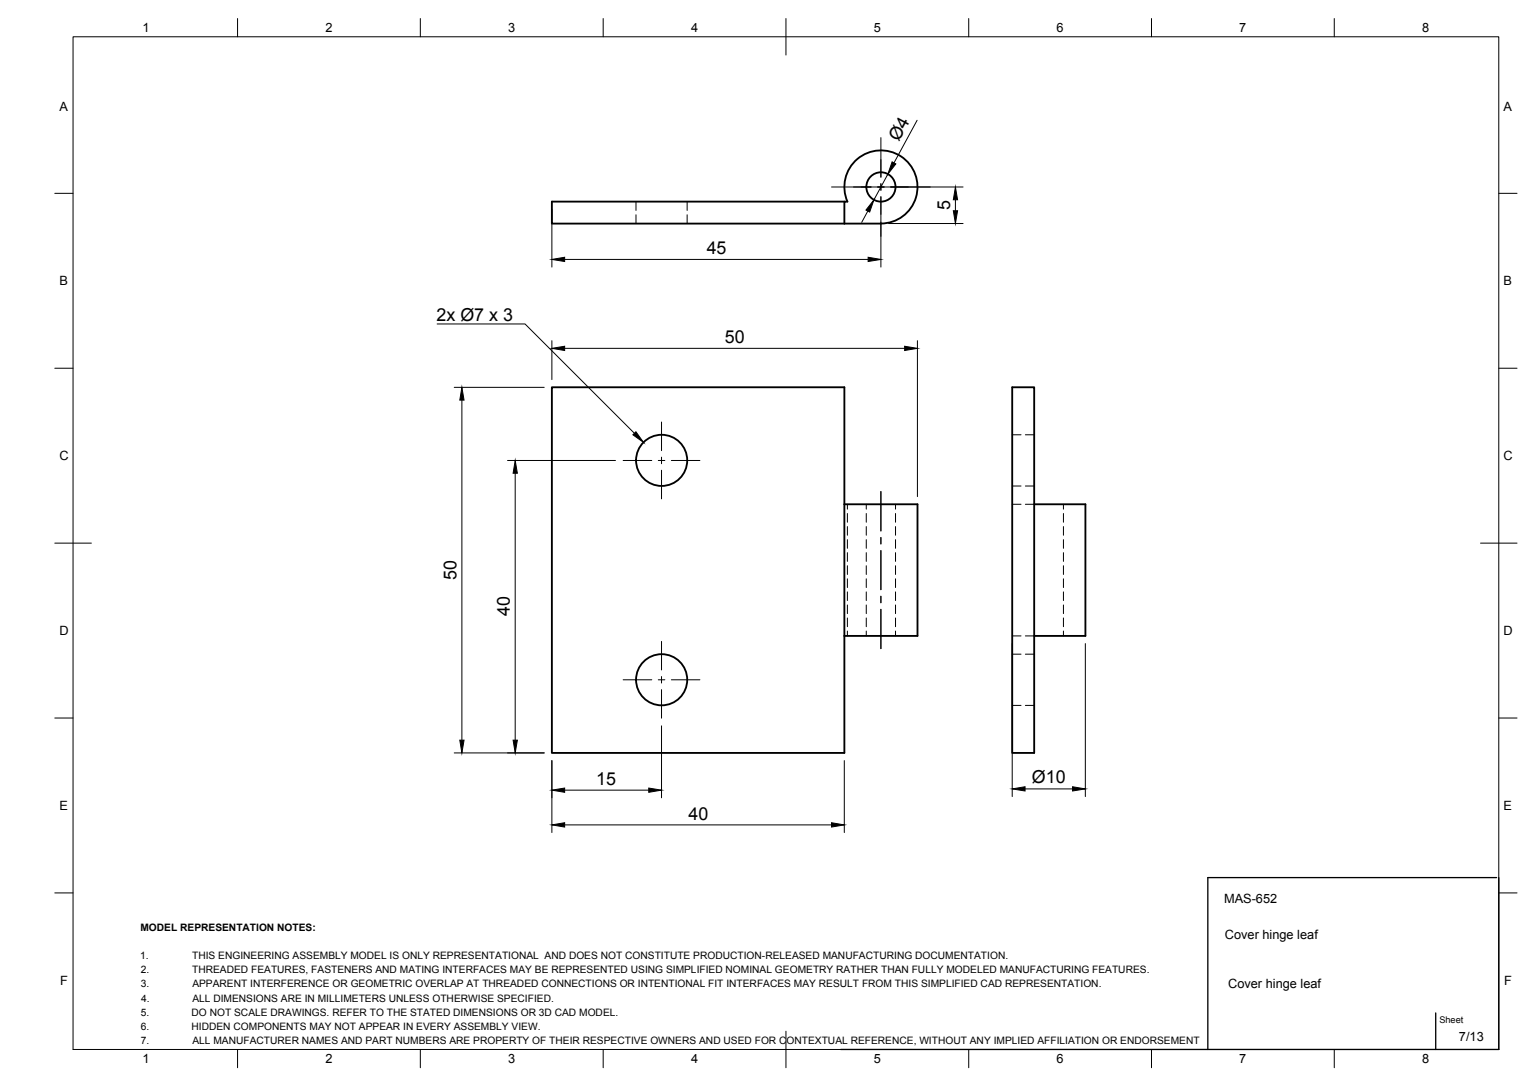
ISO-10303-21;
HEADER;
/* Generated by software containing ST-Developer
 * from STEP Tools, Inc. (www.steptools.com) 
 */

FILE_DESCRIPTION(
/* description */ ('Independent hinged machine back cover with retained hinge pins, perim
eter gasket and quarter-turn cam latch. Nominal cover 360 x 260 x 3 mm
, frame 430 x 300 x 20 mm. No guarding, structural or ingress rating a
ssigned.'),
/* implementation_level */ '2;1');

FILE_NAME(
/* name */ 'Cover hinge leaf.step',
/* time_stamp */ '2026-11-09T19:36:59-08:00',
/* author */ (''),
/* organization */ (''),
/* preprocessor_version */ 'ST-DEVELOPER v20.2',
/* originating_system */ 'Autodesk Translation Framework v15.17.0.0',
/* authorisation */ '');

FILE_SCHEMA (('AUTOMOTIVE_DESIGN { 1 0 10303 214 3 1 1 }'));
ENDSEC;

DATA;
#10=MECHANICAL_DESIGN_GEOMETRIC_PRESENTATION_REPRESENTATION('',(#210),#32627);
#174=SHAPE_REPRESENTATION_RELATIONSHIP('SRR','None',#32720,#192);
#192=ADVANCED_BREP_SHAPE_REPRESENTATION('',(#228),#32621);
#210=STYLED_ITEM('',(#32811),#228);
#228=MANIFOLD_SOLID_BREP('Body1',#8687);
#277=FACE_BOUND('',#1313,.T.);
#278=FACE_BOUND('',#1314,.T.);
#279=FACE_BOUND('',#1319,.T.);
#280=FACE_BOUND('',#1323,.T.);
#281=FACE_BOUND('',#1327,.T.);
#282=FACE_BOUND('',#1328,.T.);
#411=PLANE('',#9324);
#412=PLANE('',#9325);
#413=PLANE('',#9326);
#414=PLANE('',#9329);
#415=PLANE('',#9334);
#416=PLANE('',#9341);
#417=PLANE('',#9342);
#418=PLANE('',#9343);
#419=PLANE('',#9344);
#792=FACE_OUTER_BOUND('',#1310,.T.);
#793=FACE_OUTER_BOUND('',#1311,.T.);
#794=FACE_OUTER_BOUND('',#1312,.T.);
#795=FACE_OUTER_BOUND('',#1315,.T.);
#796=FACE_OUTER_BOUND('',#1316,.T.);
#797=FACE_OUTER_BOUND('',#1317,.T.);
#798=FACE_OUTER_BOUND('',#1318,.T.);
#799=FACE_OUTER_BOUND('',#1320,.T.);
#800=FACE_OUTER_BOUND('',#1321,.T.);
#801=FACE_OUTER_BOUND('',#1322,.T.);
#802=FACE_OUTER_BOUND('',#1324,.T.);
#803=FACE_OUTER_BOUND('',#1325,.T.);
#804=FACE_OUTER_BOUND('',#1326,.T.);
#1310=EDGE_LOOP('',(#7173,#7174,#7175,#7176));
#1311=EDGE_LOOP('',(#7177,#7178,#7179,#7180));
#1312=EDGE_LOOP('',(#7181,#7182,#7183,#7184,#7185,#7186,#7187,#7188));
#1313=EDGE_LOOP('',(#7189));
#1314=EDGE_LOOP('',(#7190));
#1315=EDGE_LOOP('',(#7191,#7192,#7193,#7194));
#1316=EDGE_LOOP('',(#7195,#7196,#7197,#7198));
#1317=EDGE_LOOP('',(#7199,#7200,#7201,#7202));
#1318=EDGE_LOOP('',(#7203,#7204,#7205,#7206));
#1319=EDGE_LOOP('',(#7207));
#1320=EDGE_LOOP('',(#7208,#7209,#7210,#7211));
#1321=EDGE_LOOP('',(#7212,#7213,#7214,#7215));
#1322=EDGE_LOOP('',(#7216,#7217,#7218,#7219));
#1323=EDGE_LOOP('',(#7220));
#1324=EDGE_LOOP('',(#7221,#7222,#7223,#7224));
#1325=EDGE_LOOP('',(#7225,#7226,#7227,#7228));
#1326=EDGE_LOOP('',(#7229,#7230,#7231,#7232,#7233,#7234,#7235,#7236));
#1327=EDGE_LOOP('',(#7237));
#1328=EDGE_LOOP('',(#7238));
#1551=CIRCLE('',#9327,3.5);
#1552=CIRCLE('',#9328,3.5);
#1553=CIRCLE('',#9331,3.5);
#1554=CIRCLE('',#9333,3.5);
#1555=CIRCLE('',#9335,5.);
#1556=CIRCLE('',#9336,2.);
#1557=CIRCLE('',#9338,2.);
#1558=CIRCLE('',#9340,5.);
#2564=LINE('',#26316,#3110);
#2565=LINE('',#26318,#3111);
#2566=LINE('',#26320,#3112);
#2567=LINE('',#26321,#3113);
#2568=LINE('',#26325,#3114);
#2569=LINE('',#26327,#3115);
#2570=LINE('',#26329,#3116);
#2571=LINE('',#26330,#3117);
#2572=LINE('',#26333,#3118);
#2573=LINE('',#26335,#3119);
#2574=LINE('',#26336,#3120);
#2575=LINE('',#26338,#3121);
#2576=LINE('',#26340,#3122);
#2577=LINE('',#26341,#3123);
#2578=LINE('',#26348,#3124);
#2579=LINE('',#26349,#3125);
#2580=LINE('',#26353,#3126);
#2581=LINE('',#26357,#3127);
#2582=LINE('',#26361,#3128);
#2583=LINE('',#26366,#3129);
#2584=LINE('',#26370,#3130);
#2585=LINE('',#26373,#3131);
#2586=LINE('',#26376,#3132);
#2587=LINE('',#26377,#3133);
#2588=LINE('',#26379,#3134);
#3110=VECTOR('',#10784,10.);
#3111=VECTOR('',#10785,10.);
#3112=VECTOR('',#10786,10.);
#3113=VECTOR('',#10787,10.);
#3114=VECTOR('',#10790,10.);
#3115=VECTOR('',#10791,10.);
#3116=VECTOR('',#10792,10.);
#3117=VECTOR('',#10793,10.);
#3118=VECTOR('',#10796,10.);
#3119=VECTOR('',#10797,10.);
#3120=VECTOR('',#10798,10.);
#3121=VECTOR('',#10799,10.);
#3122=VECTOR('',#10800,10.);
#3123=VECTOR('',#10801,10.);
#3124=VECTOR('',#10808,10.);
#3125=VECTOR('',#10809,10.);
#3126=VECTOR('',#10814,3.5);
#3127=VECTOR('',#10819,3.5);
#3128=VECTOR('',#10824,10.);
#3129=VECTOR('',#10829,2.);
#3130=VECTOR('',#10834,10.);
#3131=VECTOR('',#10839,10.);
#3132=VECTOR('',#10842,10.);
#3133=VECTOR('',#10843,10.);
#3134=VECTOR('',#10846,10.);
#3869=VERTEX_POINT('',#26314);
#3870=VERTEX_POINT('',#26315);
#3871=VERTEX_POINT('',#26317);
#3872=VERTEX_POINT('',#26319);
#3873=VERTEX_POINT('',#26323);
#3874=VERTEX_POINT('',#26324);
#3875=VERTEX_POINT('',#26326);
#3876=VERTEX_POINT('',#26328);
#3877=VERTEX_POINT('',#26332);
#3878=VERTEX_POINT('',#26334);
#3879=VERTEX_POINT('',#26337);
#3880=VERTEX_POINT('',#26339);
#3881=VERTEX_POINT('',#26342);
#3882=VERTEX_POINT('',#26344);
#3883=VERTEX_POINT('',#26347);
#3884=VERTEX_POINT('',#26351);
#3885=VERTEX_POINT('',#26355);
#3886=VERTEX_POINT('',#26359);
#3887=VERTEX_POINT('',#26362);
#3888=VERTEX_POINT('',#26365);
#3889=VERTEX_POINT('',#26369);
#3890=VERTEX_POINT('',#26375);
#5010=EDGE_CURVE('',#3869,#3870,#2564,.T.);
#5011=EDGE_CURVE('',#3869,#3871,#2565,.T.);
#5012=EDGE_CURVE('',#3872,#3871,#2566,.T.);
#5013=EDGE_CURVE('',#3870,#3872,#2567,.T.);
#5014=EDGE_CURVE('',#3873,#3874,#2568,.T.);
#5015=EDGE_CURVE('',#3875,#3873,#2569,.T.);
#5016=EDGE_CURVE('',#3876,#3875,#2570,.T.);
#5017=EDGE_CURVE('',#3874,#3876,#2571,.T.);
#5018=EDGE_CURVE('',#3871,#3877,#2572,.T.);
#5019=EDGE_CURVE('',#3877,#3878,#2573,.T.);
#5020=EDGE_CURVE('',#3878,#3876,#2574,.T.);
#5021=EDGE_CURVE('',#3879,#3875,#2575,.T.);
#5022=EDGE_CURVE('',#3880,#3879,#2576,.T.);
#5023=EDGE_CURVE('',#3872,#3880,#2577,.T.);
#5024=EDGE_CURVE('',#3881,#3881,#1551,.T.);
#5025=EDGE_CURVE('',#3882,#3882,#1552,.T.);
#5026=EDGE_CURVE('',#3883,#3873,#2578,.T.);
#5027=EDGE_CURVE('',#3879,#3883,#2579,.T.);
#5028=EDGE_CURVE('',#3884,#3884,#1553,.T.);
#5029=EDGE_CURVE('',#3884,#3882,#2580,.T.);
#5030=EDGE_CURVE('',#3885,#3885,#1554,.T.);
#5031=EDGE_CURVE('',#3885,#3881,#2581,.T.);
#5032=EDGE_CURVE('',#3878,#3886,#1555,.T.);
#5033=EDGE_CURVE('',#3874,#3886,#2582,.T.);
#5034=EDGE_CURVE('',#3887,#3887,#1556,.T.);
#5035=EDGE_CURVE('',#3887,#3888,#2583,.T.);
#5036=EDGE_CURVE('',#3888,#3888,#1557,.T.);
#5037=EDGE_CURVE('',#3886,#3889,#2584,.T.);
#5038=EDGE_CURVE('',#3877,#3889,#1558,.T.);
#5039=EDGE_CURVE('',#3889,#3869,#2585,.T.);
#5040=EDGE_CURVE('',#3890,#3883,#2586,.T.);
#5041=EDGE_CURVE('',#3880,#3890,#2587,.T.);
#5042=EDGE_CURVE('',#3870,#3890,#2588,.T.);
#7173=ORIENTED_EDGE('',*,*,#5010,.F.);
#7174=ORIENTED_EDGE('',*,*,#5011,.T.);
#7175=ORIENTED_EDGE('',*,*,#5012,.F.);
#7176=ORIENTED_EDGE('',*,*,#5013,.F.);
#7177=ORIENTED_EDGE('',*,*,#5014,.F.);
#7178=ORIENTED_EDGE('',*,*,#5015,.F.);
#7179=ORIENTED_EDGE('',*,*,#5016,.F.);
#7180=ORIENTED_EDGE('',*,*,#5017,.F.);
#7181=ORIENTED_EDGE('',*,*,#5012,.T.);
#7182=ORIENTED_EDGE('',*,*,#5018,.T.);
#7183=ORIENTED_EDGE('',*,*,#5019,.T.);
#7184=ORIENTED_EDGE('',*,*,#5020,.T.);
#7185=ORIENTED_EDGE('',*,*,#5016,.T.);
#7186=ORIENTED_EDGE('',*,*,#5021,.F.);
#7187=ORIENTED_EDGE('',*,*,#5022,.F.);
#7188=ORIENTED_EDGE('',*,*,#5023,.F.);
#7189=ORIENTED_EDGE('',*,*,#5024,.T.);
#7190=ORIENTED_EDGE('',*,*,#5025,.T.);
#7191=ORIENTED_EDGE('',*,*,#5015,.T.);
#7192=ORIENTED_EDGE('',*,*,#5026,.F.);
#7193=ORIENTED_EDGE('',*,*,#5027,.F.);
#7194=ORIENTED_EDGE('',*,*,#5021,.T.);
#7195=ORIENTED_EDGE('',*,*,#5028,.F.);
#7196=ORIENTED_EDGE('',*,*,#5029,.T.);
#7197=ORIENTED_EDGE('',*,*,#5025,.F.);
#7198=ORIENTED_EDGE('',*,*,#5029,.F.);
#7199=ORIENTED_EDGE('',*,*,#5030,.F.);
#7200=ORIENTED_EDGE('',*,*,#5031,.T.);
#7201=ORIENTED_EDGE('',*,*,#5024,.F.);
#7202=ORIENTED_EDGE('',*,*,#5031,.F.);
#7203=ORIENTED_EDGE('',*,*,#5032,.T.);
#7204=ORIENTED_EDGE('',*,*,#5033,.F.);
#7205=ORIENTED_EDGE('',*,*,#5017,.T.);
#7206=ORIENTED_EDGE('',*,*,#5020,.F.);
#7207=ORIENTED_EDGE('',*,*,#5034,.T.);
#7208=ORIENTED_EDGE('',*,*,#5034,.F.);
#7209=ORIENTED_EDGE('',*,*,#5035,.T.);
#7210=ORIENTED_EDGE('',*,*,#5036,.T.);
#7211=ORIENTED_EDGE('',*,*,#5035,.F.);
#7212=ORIENTED_EDGE('',*,*,#5037,.F.);
#7213=ORIENTED_EDGE('',*,*,#5032,.F.);
#7214=ORIENTED_EDGE('',*,*,#5019,.F.);
#7215=ORIENTED_EDGE('',*,*,#5038,.T.);
#7216=ORIENTED_EDGE('',*,*,#5018,.F.);
#7217=ORIENTED_EDGE('',*,*,#5011,.F.);
#7218=ORIENTED_EDGE('',*,*,#5039,.F.);
#7219=ORIENTED_EDGE('',*,*,#5038,.F.);
#7220=ORIENTED_EDGE('',*,*,#5036,.F.);
#7221=ORIENTED_EDGE('',*,*,#5022,.T.);
#7222=ORIENTED_EDGE('',*,*,#5027,.T.);
#7223=ORIENTED_EDGE('',*,*,#5040,.F.);
#7224=ORIENTED_EDGE('',*,*,#5041,.F.);
#7225=ORIENTED_EDGE('',*,*,#5013,.T.);
#7226=ORIENTED_EDGE('',*,*,#5023,.T.);
#7227=ORIENTED_EDGE('',*,*,#5041,.T.);
#7228=ORIENTED_EDGE('',*,*,#5042,.F.);
#7229=ORIENTED_EDGE('',*,*,#5010,.T.);
#7230=ORIENTED_EDGE('',*,*,#5042,.T.);
#7231=ORIENTED_EDGE('',*,*,#5040,.T.);
#7232=ORIENTED_EDGE('',*,*,#5026,.T.);
#7233=ORIENTED_EDGE('',*,*,#5014,.T.);
#7234=ORIENTED_EDGE('',*,*,#5033,.T.);
#7235=ORIENTED_EDGE('',*,*,#5037,.T.);
#7236=ORIENTED_EDGE('',*,*,#5039,.T.);
#7237=ORIENTED_EDGE('',*,*,#5028,.T.);
#7238=ORIENTED_EDGE('',*,*,#5030,.T.);
#8114=CYLINDRICAL_SURFACE('',#9330,3.5);
#8115=CYLINDRICAL_SURFACE('',#9332,3.5);
#8116=CYLINDRICAL_SURFACE('',#9337,2.);
#8117=CYLINDRICAL_SURFACE('',#9339,5.);
#8540=ADVANCED_FACE('',(#792),#411,.F.);
#8541=ADVANCED_FACE('',(#793),#412,.F.);
#8542=ADVANCED_FACE('',(#794,#277,#278),#413,.F.);
#8543=ADVANCED_FACE('',(#795),#414,.T.);
#8544=ADVANCED_FACE('',(#796),#8114,.F.);
#8545=ADVANCED_FACE('',(#797),#8115,.F.);
#8546=ADVANCED_FACE('',(#798,#279),#415,.T.);
#8547=ADVANCED_FACE('',(#799),#8116,.F.);
#8548=ADVANCED_FACE('',(#800),#8117,.T.);
#8549=ADVANCED_FACE('',(#801,#280),#416,.F.);
#8550=ADVANCED_FACE('',(#802),#417,.T.);
#8551=ADVANCED_FACE('',(#803),#418,.T.);
#8552=ADVANCED_FACE('',(#804,#281,#282),#419,.T.);
#8687=CLOSED_SHELL('',(#8540,#8541,#8542,#8543,#8544,#8545,#8546,#8547,
#8548,#8549,#8550,#8551,#8552));
#9323=AXIS2_PLACEMENT_3D('',#26312,#10780,#10781);
#9324=AXIS2_PLACEMENT_3D('',#26313,#10782,#10783);
#9325=AXIS2_PLACEMENT_3D('',#26322,#10788,#10789);
#9326=AXIS2_PLACEMENT_3D('',#26331,#10794,#10795);
#9327=AXIS2_PLACEMENT_3D('',#26343,#10802,#10803);
#9328=AXIS2_PLACEMENT_3D('',#26345,#10804,#10805);
#9329=AXIS2_PLACEMENT_3D('',#26346,#10806,#10807);
#9330=AXIS2_PLACEMENT_3D('',#26350,#10810,#10811);
#9331=AXIS2_PLACEMENT_3D('',#26352,#10812,#10813);
#9332=AXIS2_PLACEMENT_3D('',#26354,#10815,#10816);
#9333=AXIS2_PLACEMENT_3D('',#26356,#10817,#10818);
#9334=AXIS2_PLACEMENT_3D('',#26358,#10820,#10821);
#9335=AXIS2_PLACEMENT_3D('',#26360,#10822,#10823);
#9336=AXIS2_PLACEMENT_3D('',#26363,#10825,#10826);
#9337=AXIS2_PLACEMENT_3D('',#26364,#10827,#10828);
#9338=AXIS2_PLACEMENT_3D('',#26367,#10830,#10831);
#9339=AXIS2_PLACEMENT_3D('',#26368,#10832,#10833);
#9340=AXIS2_PLACEMENT_3D('',#26371,#10835,#10836);
#9341=AXIS2_PLACEMENT_3D('',#26372,#10837,#10838);
#9342=AXIS2_PLACEMENT_3D('',#26374,#10840,#10841);
#9343=AXIS2_PLACEMENT_3D('',#26378,#10844,#10845);
#9344=AXIS2_PLACEMENT_3D('',#26380,#10847,#10848);
#10780=DIRECTION('axis',(0.,0.,1.));
#10781=DIRECTION('refdir',(1.,0.,0.));
#10782=DIRECTION('center_axis',(1.,0.,0.));
#10783=DIRECTION('ref_axis',(0.,-1.,0.));
#10784=DIRECTION('',(0.,-1.,0.));
#10785=DIRECTION('',(0.,0.,-1.));
#10786=DIRECTION('',(0.,1.,0.));
#10787=DIRECTION('',(0.,0.,-1.));
#10788=DIRECTION('center_axis',(1.,0.,0.));
#10789=DIRECTION('ref_axis',(0.,-1.,0.));
#10790=DIRECTION('',(0.,-1.,0.));
#10791=DIRECTION('',(0.,0.,1.));
#10792=DIRECTION('',(0.,1.,0.));
#10793=DIRECTION('',(0.,0.,-1.));
#10794=DIRECTION('center_axis',(0.,0.,1.));
#10795=DIRECTION('ref_axis',(1.,0.,0.));
#10796=DIRECTION('',(-1.,0.,0.));
#10797=DIRECTION('',(0.,1.,0.));
#10798=DIRECTION('',(1.,0.,0.));
#10799=DIRECTION('',(-1.,0.,0.));
#10800=DIRECTION('',(0.,1.,0.));
#10801=DIRECTION('',(1.,0.,0.));
#10802=DIRECTION('center_axis',(0.,0.,1.));
#10803=DIRECTION('ref_axis',(1.,0.,0.));
#10804=DIRECTION('center_axis',(0.,0.,1.));
#10805=DIRECTION('ref_axis',(1.,0.,0.));
#10806=DIRECTION('center_axis',(0.,1.,0.));
#10807=DIRECTION('ref_axis',(-1.,0.,0.));
#10808=DIRECTION('',(-1.,0.,0.));
#10809=DIRECTION('',(0.,0.,1.));
#10810=DIRECTION('center_axis',(0.,0.,-1.));
#10811=DIRECTION('ref_axis',(1.,0.,0.));
#10812=DIRECTION('center_axis',(0.,0.,-1.));
#10813=DIRECTION('ref_axis',(1.,0.,0.));
#10814=DIRECTION('',(0.,0.,-1.));
#10815=DIRECTION('center_axis',(0.,0.,-1.));
#10816=DIRECTION('ref_axis',(1.,0.,0.));
#10817=DIRECTION('center_axis',(0.,0.,-1.));
#10818=DIRECTION('ref_axis',(1.,0.,0.));
#10819=DIRECTION('',(0.,0.,-1.));
#10820=DIRECTION('center_axis',(0.,1.,0.));
#10821=DIRECTION('ref_axis',(1.,0.,0.));
#10822=DIRECTION('center_axis',(0.,1.,0.));
#10823=DIRECTION('ref_axis',(1.,0.,0.));
#10824=DIRECTION('',(-1.,0.,0.));
#10825=DIRECTION('center_axis',(0.,-1.,0.));
#10826=DIRECTION('ref_axis',(1.,0.,0.));
#10827=DIRECTION('center_axis',(0.,1.,0.));
#10828=DIRECTION('ref_axis',(1.,0.,0.));
#10829=DIRECTION('',(0.,-1.,0.));
#10830=DIRECTION('center_axis',(0.,-1.,0.));
#10831=DIRECTION('ref_axis',(1.,0.,0.));
#10832=DIRECTION('center_axis',(0.,1.,0.));
#10833=DIRECTION('ref_axis',(-0.547722557505167,0.,-0.836660026534075));
#10834=DIRECTION('',(0.,-1.,0.));
#10835=DIRECTION('center_axis',(0.,1.,0.));
#10836=DIRECTION('ref_axis',(1.,0.,0.));
#10837=DIRECTION('center_axis',(0.,1.,0.));
#10838=DIRECTION('ref_axis',(1.,0.,0.));
#10839=DIRECTION('',(1.,0.,0.));
#10840=DIRECTION('center_axis',(1.,0.,0.));
#10841=DIRECTION('ref_axis',(0.,1.,0.));
#10842=DIRECTION('',(0.,1.,0.));
#10843=DIRECTION('',(0.,0.,1.));
#10844=DIRECTION('center_axis',(0.,-1.,0.));
#10845=DIRECTION('ref_axis',(1.,0.,0.));
#10846=DIRECTION('',(1.,0.,0.));
#10847=DIRECTION('center_axis',(0.,0.,1.));
#10848=DIRECTION('ref_axis',(1.,0.,0.));
#26312=CARTESIAN_POINT('',(0.,0.,0.));
#26313=CARTESIAN_POINT('Origin',(5.,-9.,0.));
#26314=CARTESIAN_POINT('',(5.,-9.,0.));
#26315=CARTESIAN_POINT('',(5.,-25.,0.));
#26316=CARTESIAN_POINT('',(5.,-4.5,0.));
#26317=CARTESIAN_POINT('',(5.,-9.,-3.));
#26318=CARTESIAN_POINT('',(5.,-9.,0.));
#26319=CARTESIAN_POINT('',(5.,-25.,-3.));
#26320=CARTESIAN_POINT('',(5.,-4.5,-3.));
#26321=CARTESIAN_POINT('',(5.,-25.,-1.5));
#26322=CARTESIAN_POINT('Origin',(5.,25.,0.));
#26323=CARTESIAN_POINT('',(5.,25.,0.));
#26324=CARTESIAN_POINT('',(5.,9.,0.));
#26325=CARTESIAN_POINT('',(5.,12.5,0.));
#26326=CARTESIAN_POINT('',(5.,25.,-3.));
#26327=CARTESIAN_POINT('',(5.,25.,-1.5));
#26328=CARTESIAN_POINT('',(5.,9.,-3.));
#26329=CARTESIAN_POINT('',(5.,12.5,-3.));
#26330=CARTESIAN_POINT('',(5.,9.,0.));
#26331=CARTESIAN_POINT('Origin',(22.5,0.,-3.));
#26332=CARTESIAN_POINT('',(4.58257569495584,-9.,-3.));
#26333=CARTESIAN_POINT('',(11.25,-9.,-3.));
#26334=CARTESIAN_POINT('',(4.58257569495584,9.,-3.));
#26335=CARTESIAN_POINT('',(4.58257569495584,-9.,-3.));
#26336=CARTESIAN_POINT('',(13.75,9.,-3.));
#26337=CARTESIAN_POINT('',(45.,25.,-3.));
#26338=CARTESIAN_POINT('',(45.,25.,-3.));
#26339=CARTESIAN_POINT('',(45.,-25.,-3.));
#26340=CARTESIAN_POINT('',(45.,-25.,-3.));
#26341=CARTESIAN_POINT('',(0.,-25.,-3.));
#26342=CARTESIAN_POINT('',(26.5,15.,-3.));
#26343=CARTESIAN_POINT('Origin',(30.,15.,-3.));
#26344=CARTESIAN_POINT('',(26.5,-15.,-3.));
#26345=CARTESIAN_POINT('Origin',(30.,-15.,-3.));
#26346=CARTESIAN_POINT('Origin',(45.,25.,-3.));
#26347=CARTESIAN_POINT('',(45.,25.,0.));
#26348=CARTESIAN_POINT('',(45.,25.,0.));
#26349=CARTESIAN_POINT('',(45.,25.,-3.));
#26350=CARTESIAN_POINT('Origin',(30.,-15.,-1.5));
#26351=CARTESIAN_POINT('',(26.5,-15.,0.));
#26352=CARTESIAN_POINT('Origin',(30.,-15.,0.));
#26353=CARTESIAN_POINT('',(26.5,-15.,-1.5));
#26354=CARTESIAN_POINT('Origin',(30.,15.,-1.5));
#26355=CARTESIAN_POINT('',(26.5,15.,0.));
#26356=CARTESIAN_POINT('Origin',(30.,15.,0.));
#26357=CARTESIAN_POINT('',(26.5,15.,-1.5));
#26358=CARTESIAN_POINT('Origin',(0.,9.,-5.));
#26359=CARTESIAN_POINT('',(0.,9.,0.));
#26360=CARTESIAN_POINT('Origin',(0.,9.,-5.));
#26361=CARTESIAN_POINT('',(13.75,9.,0.));
#26362=CARTESIAN_POINT('',(-2.,9.,-5.));
#26363=CARTESIAN_POINT('Origin',(0.,9.,-5.));
#26364=CARTESIAN_POINT('Origin',(0.,-9.,-5.));
#26365=CARTESIAN_POINT('',(-2.,-9.,-5.));
#26366=CARTESIAN_POINT('',(-2.,-9.,-5.));
#26367=CARTESIAN_POINT('Origin',(0.,-9.,-5.));
#26368=CARTESIAN_POINT('Origin',(0.,-9.,-5.));
#26369=CARTESIAN_POINT('',(0.,-9.,0.));
#26370=CARTESIAN_POINT('',(0.,25.,0.));
#26371=CARTESIAN_POINT('Origin',(0.,-9.,-5.));
#26372=CARTESIAN_POINT('Origin',(0.,-9.,-5.));
#26373=CARTESIAN_POINT('',(11.25,-9.,0.));
#26374=CARTESIAN_POINT('Origin',(45.,-25.,-3.));
#26375=CARTESIAN_POINT('',(45.,-25.,0.));
#26376=CARTESIAN_POINT('',(45.,-25.,0.));
#26377=CARTESIAN_POINT('',(45.,-25.,-3.));
#26378=CARTESIAN_POINT('Origin',(0.,-25.,-3.));
#26379=CARTESIAN_POINT('',(0.,-25.,0.));
#26380=CARTESIAN_POINT('Origin',(22.5,0.,0.));
#32601=UNCERTAINTY_MEASURE_WITH_UNIT(LENGTH_MEASURE(0.01),#32628,
'DISTANCE_ACCURACY_VALUE',
'Maximum model space distance between geometric entities at asserted c
onnectivities');
#32607=UNCERTAINTY_MEASURE_WITH_UNIT(LENGTH_MEASURE(0.01),#32628,
'DISTANCE_ACCURACY_VALUE',
'Maximum model space distance between geometric entities at asserted c
onnectivities');
#32621=(
GEOMETRIC_REPRESENTATION_CONTEXT(3)
GLOBAL_UNCERTAINTY_ASSIGNED_CONTEXT((#32601))
GLOBAL_UNIT_ASSIGNED_CONTEXT((#32628,#32630,#32631))
REPRESENTATION_CONTEXT('','3D')
);
#32627=(
GEOMETRIC_REPRESENTATION_CONTEXT(3)
GLOBAL_UNCERTAINTY_ASSIGNED_CONTEXT((#32607))
GLOBAL_UNIT_ASSIGNED_CONTEXT((#32628,#32630,#32631))
REPRESENTATION_CONTEXT('','3D')
);
#32628=(
LENGTH_UNIT()
NAMED_UNIT(*)
SI_UNIT(.MILLI.,.METRE.)
);
#32630=(
NAMED_UNIT(*)
PLANE_ANGLE_UNIT()
SI_UNIT($,.RADIAN.)
);
#32631=(
NAMED_UNIT(*)
SI_UNIT($,.STERADIAN.)
SOLID_ANGLE_UNIT()
);
#32645=SHAPE_DEFINITION_REPRESENTATION(#32664,#32720);
#32664=PRODUCT_DEFINITION_SHAPE('',$,#32740);
#32720=SHAPE_REPRESENTATION('',(#9323),#32621);
#32726=PRODUCT_DEFINITION_CONTEXT('part definition',#32785,'design');
#32740=PRODUCT_DEFINITION('Cover hinge leaf','Cover hinge leaf',#32759,
#32726);
#32759=PRODUCT_DEFINITION_FORMATION('',$,#32800);
#32785=APPLICATION_CONTEXT(
'Core Data for Automotive Mechanical Design Process');
#32786=PRODUCT_CONTEXT('part definition',#32785,'mechanical');
#32800=PRODUCT('Cover hinge leaf','Cover hinge leaf',$,(#32786));
#32811=PRESENTATION_STYLE_ASSIGNMENT((#32818));
#32818=SURFACE_STYLE_USAGE(.BOTH.,#32825);
#32825=SURFACE_SIDE_STYLE('',(#32832));
#32832=SURFACE_STYLE_FILL_AREA(#32839);
#32839=FILL_AREA_STYLE('Sky blue',(#32846));
#32846=FILL_AREA_STYLE_COLOUR('Sky blue',#32853);
#32853=COLOUR_RGB('Sky blue',0.317647058823529,0.686274509803922,0.890196078431372);
ENDSEC;
END-ISO-10303-21;
